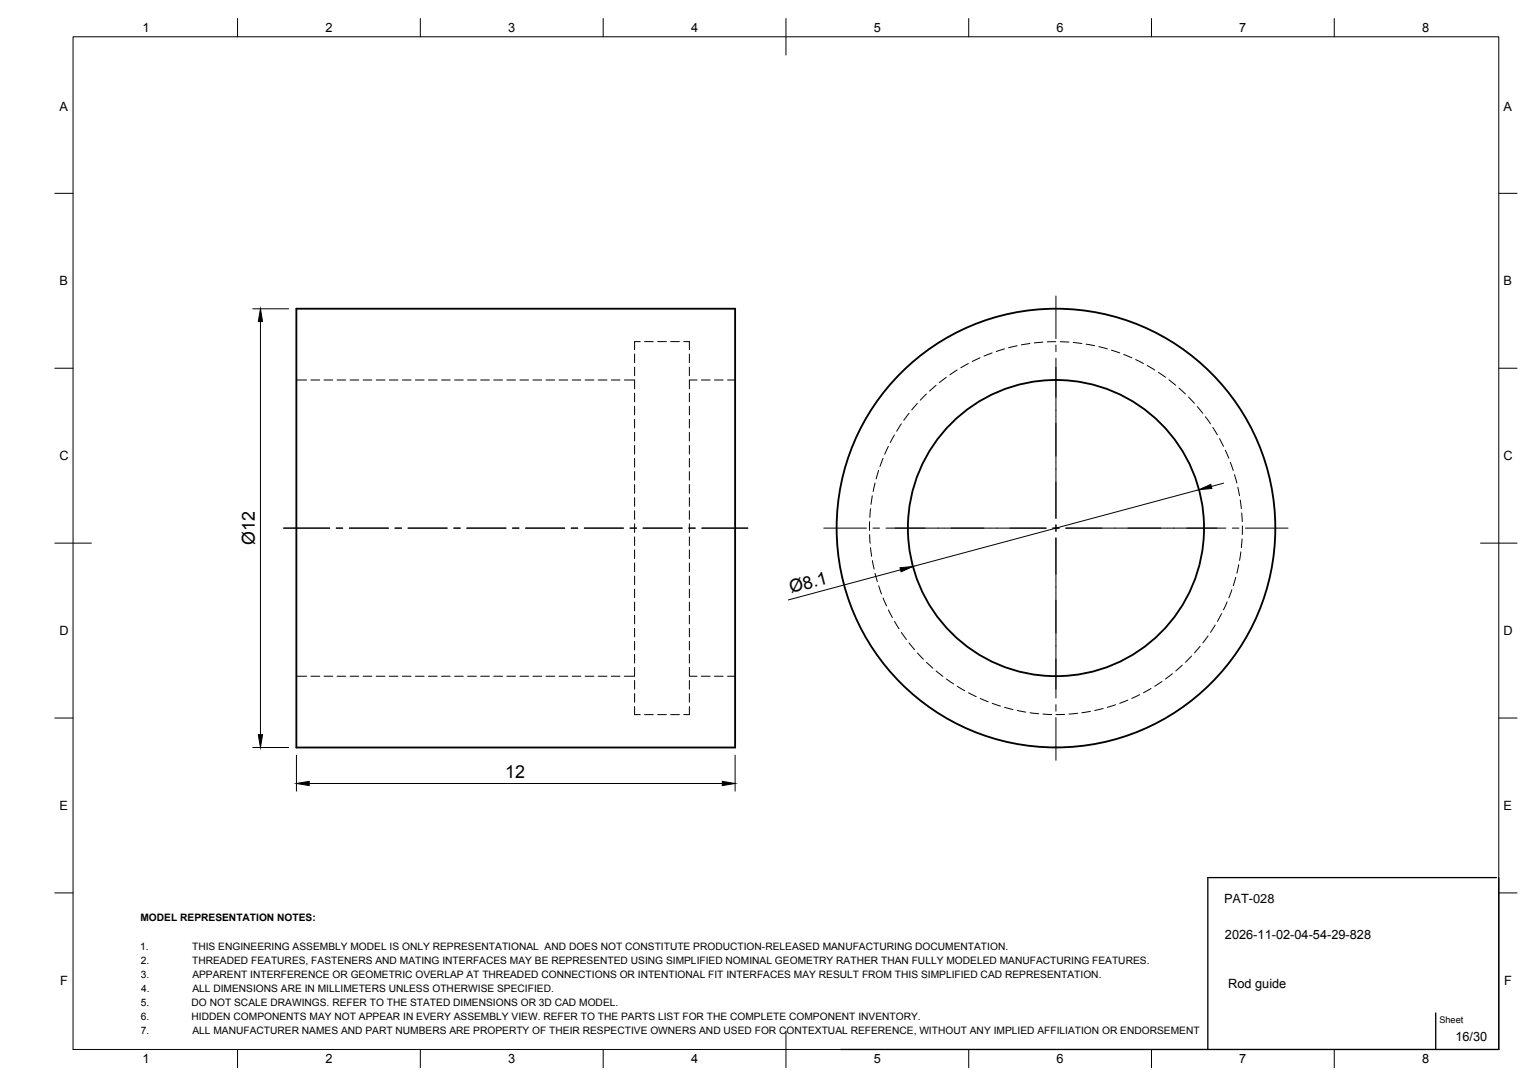
ISO-10303-21;
HEADER;
/* Generated by software containing ST-Developer
 * from STEP Tools, Inc. (www.steptools.com) 
 */

FILE_DESCRIPTION(
/* description */ ('Cylinder foot and clevis mount kit'),
/* implementation_level */ '2;1');

FILE_NAME(
/* name */ 'Rod guide.step',
/* time_stamp */ '2026-10-27T20:10:43-07:00',
/* author */ (''),
/* organization */ (''),
/* preprocessor_version */ 'ST-DEVELOPER v20.2',
/* originating_system */ 'Autodesk Translation Framework v15.17.0.0',
/* authorisation */ '');

FILE_SCHEMA (('AUTOMOTIVE_DESIGN { 1 0 10303 214 3 1 1 }'));
ENDSEC;

DATA;
#10=MECHANICAL_DESIGN_GEOMETRIC_PRESENTATION_REPRESENTATION('',(#352),#9102);
#296=SHAPE_REPRESENTATION_RELATIONSHIP('SRR','None',#9244,#324);
#324=ADVANCED_BREP_SHAPE_REPRESENTATION('',(#379),#9087);
#352=STYLED_ITEM('',(#9460),#379);
#379=MANIFOLD_SOLID_BREP('Body1',#4939);
#466=FACE_BOUND('',#1277,.T.);
#467=FACE_BOUND('',#1279,.T.);
#468=FACE_BOUND('',#1284,.T.);
#469=FACE_BOUND('',#1286,.T.);
#631=PLANE('',#5646);
#632=PLANE('',#5648);
#633=PLANE('',#5657);
#634=PLANE('',#5658);
#895=FACE_OUTER_BOUND('',#1275,.T.);
#896=FACE_OUTER_BOUND('',#1276,.T.);
#897=FACE_OUTER_BOUND('',#1278,.T.);
#898=FACE_OUTER_BOUND('',#1280,.T.);
#899=FACE_OUTER_BOUND('',#1281,.T.);
#900=FACE_OUTER_BOUND('',#1282,.T.);
#901=FACE_OUTER_BOUND('',#1283,.T.);
#902=FACE_OUTER_BOUND('',#1285,.T.);
#1275=EDGE_LOOP('',(#4109,#4110,#4111,#4112));
#1276=EDGE_LOOP('',(#4113));
#1277=EDGE_LOOP('',(#4114));
#1278=EDGE_LOOP('',(#4115));
#1279=EDGE_LOOP('',(#4116));
#1280=EDGE_LOOP('',(#4117,#4118,#4119,#4120));
#1281=EDGE_LOOP('',(#4121,#4122,#4123,#4124));
#1282=EDGE_LOOP('',(#4125,#4126,#4127,#4128));
#1283=EDGE_LOOP('',(#4129));
#1284=EDGE_LOOP('',(#4130));
#1285=EDGE_LOOP('',(#4131));
#1286=EDGE_LOOP('',(#4132));
#1647=LINE('',#8368,#1996);
#1648=LINE('',#8378,#1997);
#1649=LINE('',#8383,#1998);
#1650=LINE('',#8388,#1999);
#1996=VECTOR('',#6892,0.51);
#1997=VECTOR('',#6905,0.405);
#1998=VECTOR('',#6912,0.405);
#1999=VECTOR('',#6917,0.6);
#2254=CIRCLE('',#5644,0.51);
#2255=CIRCLE('',#5645,0.51);
#2256=CIRCLE('',#5647,0.405);
#2257=CIRCLE('',#5649,0.405);
#2258=CIRCLE('',#5651,0.405);
#2259=CIRCLE('',#5653,0.405);
#2260=CIRCLE('',#5655,0.6);
#2261=CIRCLE('',#5656,0.6);
#2579=VERTEX_POINT('',#8365);
#2580=VERTEX_POINT('',#8367);
#2581=VERTEX_POINT('',#8371);
#2582=VERTEX_POINT('',#8374);
#2583=VERTEX_POINT('',#8377);
#2584=VERTEX_POINT('',#8381);
#2585=VERTEX_POINT('',#8385);
#2586=VERTEX_POINT('',#8387);
#3109=EDGE_CURVE('',#2579,#2579,#2254,.T.);
#3110=EDGE_CURVE('',#2579,#2580,#1647,.T.);
#3111=EDGE_CURVE('',#2580,#2580,#2255,.T.);
#3112=EDGE_CURVE('',#2581,#2581,#2256,.T.);
#3113=EDGE_CURVE('',#2582,#2582,#2257,.T.);
#3114=EDGE_CURVE('',#2582,#2583,#1648,.T.);
#3115=EDGE_CURVE('',#2583,#2583,#2258,.T.);
#3116=EDGE_CURVE('',#2584,#2584,#2259,.T.);
#3117=EDGE_CURVE('',#2584,#2581,#1649,.T.);
#3118=EDGE_CURVE('',#2585,#2585,#2260,.T.);
#3119=EDGE_CURVE('',#2585,#2586,#1650,.T.);
#3120=EDGE_CURVE('',#2586,#2586,#2261,.T.);
#4109=ORIENTED_EDGE('',*,*,#3109,.F.);
#4110=ORIENTED_EDGE('',*,*,#3110,.T.);
#4111=ORIENTED_EDGE('',*,*,#3111,.T.);
#4112=ORIENTED_EDGE('',*,*,#3110,.F.);
#4113=ORIENTED_EDGE('',*,*,#3111,.F.);
#4114=ORIENTED_EDGE('',*,*,#3112,.F.);
#4115=ORIENTED_EDGE('',*,*,#3109,.T.);
#4116=ORIENTED_EDGE('',*,*,#3113,.F.);
#4117=ORIENTED_EDGE('',*,*,#3113,.T.);
#4118=ORIENTED_EDGE('',*,*,#3114,.T.);
#4119=ORIENTED_EDGE('',*,*,#3115,.T.);
#4120=ORIENTED_EDGE('',*,*,#3114,.F.);
#4121=ORIENTED_EDGE('',*,*,#3116,.F.);
#4122=ORIENTED_EDGE('',*,*,#3117,.T.);
#4123=ORIENTED_EDGE('',*,*,#3112,.T.);
#4124=ORIENTED_EDGE('',*,*,#3117,.F.);
#4125=ORIENTED_EDGE('',*,*,#3118,.F.);
#4126=ORIENTED_EDGE('',*,*,#3119,.T.);
#4127=ORIENTED_EDGE('',*,*,#3120,.T.);
#4128=ORIENTED_EDGE('',*,*,#3119,.F.);
#4129=ORIENTED_EDGE('',*,*,#3118,.T.);
#4130=ORIENTED_EDGE('',*,*,#3116,.T.);
#4131=ORIENTED_EDGE('',*,*,#3120,.F.);
#4132=ORIENTED_EDGE('',*,*,#3115,.F.);
#4590=CYLINDRICAL_SURFACE('',#5643,0.51);
#4591=CYLINDRICAL_SURFACE('',#5650,0.405);
#4592=CYLINDRICAL_SURFACE('',#5652,0.405);
#4593=CYLINDRICAL_SURFACE('',#5654,0.6);
#4818=ADVANCED_FACE('',(#895),#4590,.F.);
#4819=ADVANCED_FACE('',(#896,#466),#631,.F.);
#4820=ADVANCED_FACE('',(#897,#467),#632,.T.);
#4821=ADVANCED_FACE('',(#898),#4591,.F.);
#4822=ADVANCED_FACE('',(#899),#4592,.F.);
#4823=ADVANCED_FACE('',(#900),#4593,.T.);
#4824=ADVANCED_FACE('',(#901,#468),#633,.T.);
#4825=ADVANCED_FACE('',(#902,#469),#634,.F.);
#4939=CLOSED_SHELL('',(#4818,#4819,#4820,#4821,#4822,#4823,#4824,#4825));
#5642=AXIS2_PLACEMENT_3D('',#8363,#6886,#6887);
#5643=AXIS2_PLACEMENT_3D('',#8364,#6888,#6889);
#5644=AXIS2_PLACEMENT_3D('',#8366,#6890,#6891);
#5645=AXIS2_PLACEMENT_3D('',#8369,#6893,#6894);
#5646=AXIS2_PLACEMENT_3D('',#8370,#6895,#6896);
#5647=AXIS2_PLACEMENT_3D('',#8372,#6897,#6898);
#5648=AXIS2_PLACEMENT_3D('',#8373,#6899,#6900);
#5649=AXIS2_PLACEMENT_3D('',#8375,#6901,#6902);
#5650=AXIS2_PLACEMENT_3D('',#8376,#6903,#6904);
#5651=AXIS2_PLACEMENT_3D('',#8379,#6906,#6907);
#5652=AXIS2_PLACEMENT_3D('',#8380,#6908,#6909);
#5653=AXIS2_PLACEMENT_3D('',#8382,#6910,#6911);
#5654=AXIS2_PLACEMENT_3D('',#8384,#6913,#6914);
#5655=AXIS2_PLACEMENT_3D('',#8386,#6915,#6916);
#5656=AXIS2_PLACEMENT_3D('',#8389,#6918,#6919);
#5657=AXIS2_PLACEMENT_3D('',#8390,#6920,#6921);
#5658=AXIS2_PLACEMENT_3D('',#8391,#6922,#6923);
#6886=DIRECTION('axis',(0.,0.,1.));
#6887=DIRECTION('refdir',(1.,0.,0.));
#6888=DIRECTION('center_axis',(0.,1.,0.));
#6889=DIRECTION('ref_axis',(1.,0.,0.));
#6890=DIRECTION('center_axis',(0.,1.,0.));
#6891=DIRECTION('ref_axis',(1.,0.,0.));
#6892=DIRECTION('',(0.,1.,0.));
#6893=DIRECTION('center_axis',(0.,1.,0.));
#6894=DIRECTION('ref_axis',(1.,0.,0.));
#6895=DIRECTION('center_axis',(0.,1.,0.));
#6896=DIRECTION('ref_axis',(1.,0.,0.));
#6897=DIRECTION('center_axis',(0.,-1.,0.));
#6898=DIRECTION('ref_axis',(1.,0.,0.));
#6899=DIRECTION('center_axis',(0.,1.,0.));
#6900=DIRECTION('ref_axis',(1.,0.,0.));
#6901=DIRECTION('center_axis',(0.,1.,0.));
#6902=DIRECTION('ref_axis',(1.,0.,0.));
#6903=DIRECTION('center_axis',(0.,1.,0.));
#6904=DIRECTION('ref_axis',(1.,0.,0.));
#6905=DIRECTION('',(0.,-1.,0.));
#6906=DIRECTION('center_axis',(0.,-1.,0.));
#6907=DIRECTION('ref_axis',(1.,0.,0.));
#6908=DIRECTION('center_axis',(0.,1.,0.));
#6909=DIRECTION('ref_axis',(1.,0.,0.));
#6910=DIRECTION('center_axis',(0.,-1.,0.));
#6911=DIRECTION('ref_axis',(1.,0.,0.));
#6912=DIRECTION('',(0.,-1.,0.));
#6913=DIRECTION('center_axis',(0.,1.,0.));
#6914=DIRECTION('ref_axis',(1.,0.,0.));
#6915=DIRECTION('center_axis',(0.,1.,0.));
#6916=DIRECTION('ref_axis',(1.,0.,0.));
#6917=DIRECTION('',(0.,-1.,0.));
#6918=DIRECTION('center_axis',(0.,1.,0.));
#6919=DIRECTION('ref_axis',(1.,0.,0.));
#6920=DIRECTION('center_axis',(0.,1.,0.));
#6921=DIRECTION('ref_axis',(1.,0.,0.));
#6922=DIRECTION('center_axis',(0.,1.,0.));
#6923=DIRECTION('ref_axis',(1.,0.,0.));
#8363=CARTESIAN_POINT('',(0.,0.,0.));
#8364=CARTESIAN_POINT('Origin',(0.,0.125,4.5));
#8365=CARTESIAN_POINT('',(-0.51,0.125,4.5));
#8366=CARTESIAN_POINT('Origin',(0.,0.125,4.5));
#8367=CARTESIAN_POINT('',(-0.51,0.275,4.5));
#8368=CARTESIAN_POINT('',(-0.51,0.125,4.5));
#8369=CARTESIAN_POINT('Origin',(0.,0.275,4.5));
#8370=CARTESIAN_POINT('Origin',(0.,0.275,4.5));
#8371=CARTESIAN_POINT('',(-0.405,0.275,4.5));
#8372=CARTESIAN_POINT('Origin',(0.,0.275,4.5));
#8373=CARTESIAN_POINT('Origin',(0.,0.125,4.5));
#8374=CARTESIAN_POINT('',(-0.405,0.125,4.5));
#8375=CARTESIAN_POINT('Origin',(0.,0.125,4.5));
#8376=CARTESIAN_POINT('Origin',(0.,0.,4.5));
#8377=CARTESIAN_POINT('',(-0.405,0.,4.5));
#8378=CARTESIAN_POINT('',(-0.405,0.,4.5));
#8379=CARTESIAN_POINT('Origin',(0.,0.,4.5));
#8380=CARTESIAN_POINT('Origin',(0.,0.,4.5));
#8381=CARTESIAN_POINT('',(-0.405,1.2,4.5));
#8382=CARTESIAN_POINT('Origin',(0.,1.2,4.5));
#8383=CARTESIAN_POINT('',(-0.405,0.,4.5));
#8384=CARTESIAN_POINT('Origin',(0.,0.,4.5));
#8385=CARTESIAN_POINT('',(-0.6,1.2,4.5));
#8386=CARTESIAN_POINT('Origin',(0.,1.2,4.5));
#8387=CARTESIAN_POINT('',(-0.6,0.,4.5));
#8388=CARTESIAN_POINT('',(-0.6,0.,4.5));
#8389=CARTESIAN_POINT('Origin',(0.,0.,4.5));
#8390=CARTESIAN_POINT('Origin',(0.,1.2,4.5));
#8391=CARTESIAN_POINT('Origin',(0.,0.,4.5));
#9054=UNCERTAINTY_MEASURE_WITH_UNIT(LENGTH_MEASURE(0.001),#9103,
'DISTANCE_ACCURACY_VALUE',
'Maximum model space distance between geometric entities at asserted c
onnectivities');
#9069=UNCERTAINTY_MEASURE_WITH_UNIT(LENGTH_MEASURE(0.001),#9103,
'DISTANCE_ACCURACY_VALUE',
'Maximum model space distance between geometric entities at asserted c
onnectivities');
#9087=(
GEOMETRIC_REPRESENTATION_CONTEXT(3)
GLOBAL_UNCERTAINTY_ASSIGNED_CONTEXT((#9054))
GLOBAL_UNIT_ASSIGNED_CONTEXT((#9103,#9105,#9106))
REPRESENTATION_CONTEXT('','3D')
);
#9102=(
GEOMETRIC_REPRESENTATION_CONTEXT(3)
GLOBAL_UNCERTAINTY_ASSIGNED_CONTEXT((#9069))
GLOBAL_UNIT_ASSIGNED_CONTEXT((#9103,#9105,#9106))
REPRESENTATION_CONTEXT('','3D')
);
#9103=(
LENGTH_UNIT()
NAMED_UNIT(*)
SI_UNIT(.CENTI.,.METRE.)
);
#9105=(
NAMED_UNIT(*)
PLANE_ANGLE_UNIT()
SI_UNIT($,.RADIAN.)
);
#9106=(
NAMED_UNIT(*)
SI_UNIT($,.STERADIAN.)
SOLID_ANGLE_UNIT()
);
#9124=SHAPE_DEFINITION_REPRESENTATION(#9158,#9244);
#9158=PRODUCT_DEFINITION_SHAPE('',$,#9277);
#9244=SHAPE_REPRESENTATION('',(#5642),#9087);
#9259=PRODUCT_DEFINITION_CONTEXT('part definition',#9357,'design');
#9277=PRODUCT_DEFINITION('Rod guide','Rod guide',#9309,#9259);
#9309=PRODUCT_DEFINITION_FORMATION('',$,#9376);
#9357=APPLICATION_CONTEXT(
'Core Data for Automotive Mechanical Design Process');
#9358=PRODUCT_CONTEXT('part definition',#9357,'mechanical');
#9376=PRODUCT('Rod guide','Rod guide','Rod guide',(#9358));
#9454=COLOUR_RGB('Grey',0.48,0.52,0.57);
#9455=FILL_AREA_STYLE_COLOUR('',#9454);
#9456=FILL_AREA_STYLE('',(#9455));
#9457=SURFACE_STYLE_FILL_AREA(#9456);
#9458=SURFACE_SIDE_STYLE('',(#9457));
#9459=SURFACE_STYLE_USAGE(.BOTH.,#9458);
#9460=PRESENTATION_STYLE_ASSIGNMENT((#9459));
ENDSEC;
END-ISO-10303-21;
